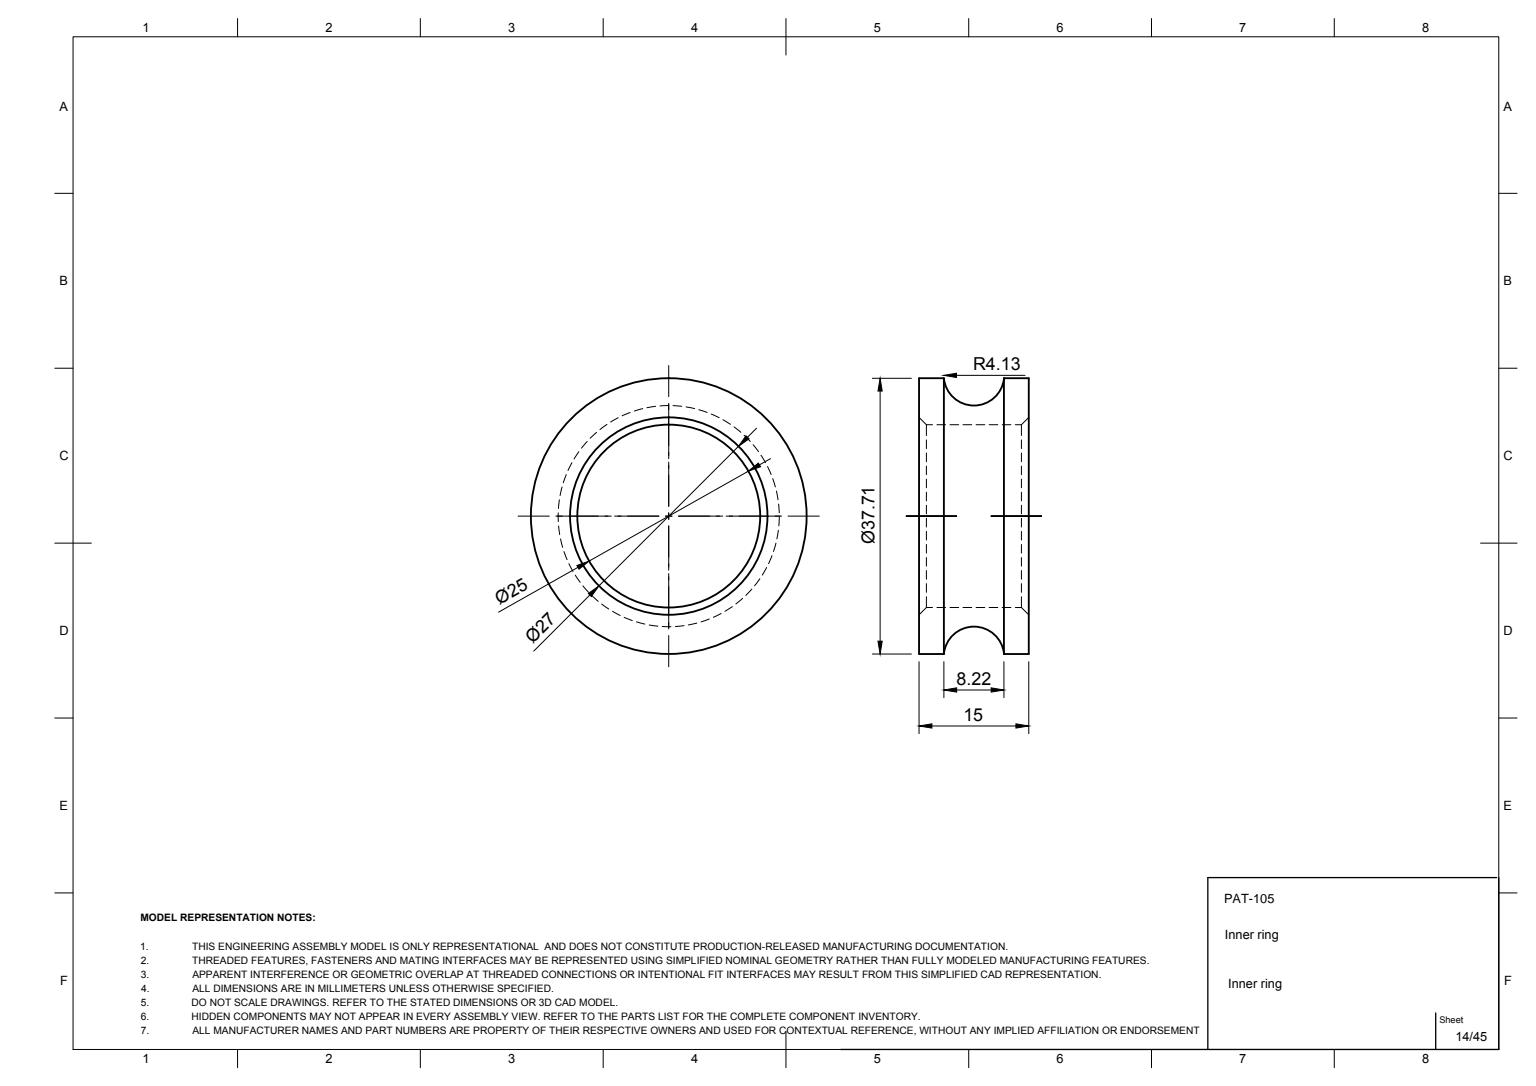
ISO-10303-21;
HEADER;
/* Generated by software containing ST-Developer
 * from STEP Tools, Inc. (www.steptools.com) 
 */

FILE_DESCRIPTION(
/* description */ ('Torque wrench calibration arm'),
/* implementation_level */ '2;1');

FILE_NAME(
/* name */ 'Inner ring.step',
/* time_stamp */ '2026-10-28T03:24:52-07:00',
/* author */ (''),
/* organization */ (''),
/* preprocessor_version */ 'ST-DEVELOPER v20.2',
/* originating_system */ 'Autodesk Translation Framework v15.17.0.0',
/* authorisation */ '');

FILE_SCHEMA (('AUTOMOTIVE_DESIGN { 1 0 10303 214 3 1 1 }'));
ENDSEC;

DATA;
#10=MECHANICAL_DESIGN_GEOMETRIC_PRESENTATION_REPRESENTATION('',(#433),#12783);
#327=CONICAL_SURFACE('',#7170,1.3,0.785398163397449);
#328=CONICAL_SURFACE('',#7177,1.3,0.785398163397449);
#348=TOROIDAL_SURFACE('',#7159,1.925,0.412776);
#359=SHAPE_REPRESENTATION_RELATIONSHIP('SRR','None',#12941,#396);
#396=ADVANCED_BREP_SHAPE_REPRESENTATION('',(#487),#12750);
#433=STYLED_ITEM('',(#13212),#487);
#487=MANIFOLD_SOLID_BREP('Body1',#6502);
#583=FACE_BOUND('',#1427,.T.);
#584=FACE_BOUND('',#1430,.T.);
#710=PLANE('',#7172);
#711=PLANE('',#7175);
#975=FACE_OUTER_BOUND('',#1422,.T.);
#976=FACE_OUTER_BOUND('',#1423,.T.);
#977=FACE_OUTER_BOUND('',#1424,.T.);
#978=FACE_OUTER_BOUND('',#1425,.T.);
#979=FACE_OUTER_BOUND('',#1426,.T.);
#980=FACE_OUTER_BOUND('',#1428,.T.);
#981=FACE_OUTER_BOUND('',#1429,.T.);
#982=FACE_OUTER_BOUND('',#1431,.T.);
#1422=EDGE_LOOP('',(#4795,#4796,#4797,#4798,#4799,#4800));
#1423=EDGE_LOOP('',(#4801,#4802,#4803,#4804,#4805));
#1424=EDGE_LOOP('',(#4806,#4807,#4808,#4809));
#1425=EDGE_LOOP('',(#4810,#4811,#4812,#4813));
#1426=EDGE_LOOP('',(#4814));
#1427=EDGE_LOOP('',(#4815));
#1428=EDGE_LOOP('',(#4816,#4817,#4818,#4819,#4820));
#1429=EDGE_LOOP('',(#4821));
#1430=EDGE_LOOP('',(#4822));
#1431=EDGE_LOOP('',(#4823,#4824,#4825,#4826));
#1920=LINE('',#10418,#2335);
#1921=LINE('',#10424,#2336);
#1922=LINE('',#10428,#2337);
#1923=LINE('',#10434,#2338);
#1924=LINE('',#10439,#2339);
#2335=VECTOR('',#8356,1.88531);
#2336=VECTOR('',#8363,1.25);
#2337=VECTOR('',#8368,1.3);
#2338=VECTOR('',#8377,1.88531);
#2339=VECTOR('',#8384,1.3);
#2704=CIRCLE('',#7160,1.88531);
#2705=CIRCLE('',#7161,1.88531);
#2706=CIRCLE('',#7162,0.412776);
#2707=CIRCLE('',#7163,1.88531);
#2708=CIRCLE('',#7164,1.88531);
#2709=CIRCLE('',#7166,1.88531);
#2710=CIRCLE('',#7168,1.25);
#2711=CIRCLE('',#7169,1.25);
#2712=CIRCLE('',#7171,1.35);
#2713=CIRCLE('',#7174,1.88531);
#2714=CIRCLE('',#7176,1.35);
#3119=VERTEX_POINT('',#10407);
#3120=VERTEX_POINT('',#10408);
#3121=VERTEX_POINT('',#10411);
#3122=VERTEX_POINT('',#10413);
#3123=VERTEX_POINT('',#10417);
#3124=VERTEX_POINT('',#10421);
#3125=VERTEX_POINT('',#10423);
#3126=VERTEX_POINT('',#10427);
#3127=VERTEX_POINT('',#10432);
#3128=VERTEX_POINT('',#10436);
#3755=EDGE_CURVE('',#3119,#3120,#2704,.T.);
#3756=EDGE_CURVE('',#3120,#3119,#2705,.T.);
#3757=EDGE_CURVE('',#3120,#3121,#2706,.T.);
#3758=EDGE_CURVE('',#3122,#3121,#2707,.T.);
#3759=EDGE_CURVE('',#3121,#3122,#2708,.T.);
#3760=EDGE_CURVE('',#3122,#3123,#1920,.T.);
#3761=EDGE_CURVE('',#3123,#3123,#2709,.T.);
#3762=EDGE_CURVE('',#3124,#3124,#2710,.T.);
#3763=EDGE_CURVE('',#3124,#3125,#1921,.T.);
#3764=EDGE_CURVE('',#3125,#3125,#2711,.T.);
#3765=EDGE_CURVE('',#3125,#3126,#1922,.T.);
#3766=EDGE_CURVE('',#3126,#3126,#2712,.T.);
#3767=EDGE_CURVE('',#3127,#3127,#2713,.T.);
#3768=EDGE_CURVE('',#3127,#3119,#1923,.T.);
#3769=EDGE_CURVE('',#3128,#3128,#2714,.T.);
#3770=EDGE_CURVE('',#3128,#3124,#1924,.T.);
#4795=ORIENTED_EDGE('',*,*,#3755,.F.);
#4796=ORIENTED_EDGE('',*,*,#3756,.F.);
#4797=ORIENTED_EDGE('',*,*,#3757,.T.);
#4798=ORIENTED_EDGE('',*,*,#3758,.F.);
#4799=ORIENTED_EDGE('',*,*,#3759,.F.);
#4800=ORIENTED_EDGE('',*,*,#3757,.F.);
#4801=ORIENTED_EDGE('',*,*,#3758,.T.);
#4802=ORIENTED_EDGE('',*,*,#3759,.T.);
#4803=ORIENTED_EDGE('',*,*,#3760,.T.);
#4804=ORIENTED_EDGE('',*,*,#3761,.T.);
#4805=ORIENTED_EDGE('',*,*,#3760,.F.);
#4806=ORIENTED_EDGE('',*,*,#3762,.T.);
#4807=ORIENTED_EDGE('',*,*,#3763,.T.);
#4808=ORIENTED_EDGE('',*,*,#3764,.F.);
#4809=ORIENTED_EDGE('',*,*,#3763,.F.);
#4810=ORIENTED_EDGE('',*,*,#3764,.T.);
#4811=ORIENTED_EDGE('',*,*,#3765,.T.);
#4812=ORIENTED_EDGE('',*,*,#3766,.F.);
#4813=ORIENTED_EDGE('',*,*,#3765,.F.);
#4814=ORIENTED_EDGE('',*,*,#3761,.F.);
#4815=ORIENTED_EDGE('',*,*,#3766,.T.);
#4816=ORIENTED_EDGE('',*,*,#3767,.F.);
#4817=ORIENTED_EDGE('',*,*,#3768,.T.);
#4818=ORIENTED_EDGE('',*,*,#3755,.T.);
#4819=ORIENTED_EDGE('',*,*,#3756,.T.);
#4820=ORIENTED_EDGE('',*,*,#3768,.F.);
#4821=ORIENTED_EDGE('',*,*,#3767,.T.);
#4822=ORIENTED_EDGE('',*,*,#3769,.F.);
#4823=ORIENTED_EDGE('',*,*,#3769,.T.);
#4824=ORIENTED_EDGE('',*,*,#3770,.T.);
#4825=ORIENTED_EDGE('',*,*,#3762,.F.);
#4826=ORIENTED_EDGE('',*,*,#3770,.F.);
#6029=CYLINDRICAL_SURFACE('',#7165,1.88531);
#6030=CYLINDRICAL_SURFACE('',#7167,1.25);
#6031=CYLINDRICAL_SURFACE('',#7173,1.88531);
#6200=ADVANCED_FACE('',(#975),#348,.F.);
#6201=ADVANCED_FACE('',(#976),#6029,.T.);
#6202=ADVANCED_FACE('',(#977),#6030,.F.);
#6203=ADVANCED_FACE('',(#978),#327,.F.);
#6204=ADVANCED_FACE('',(#979,#583),#710,.T.);
#6205=ADVANCED_FACE('',(#980),#6031,.T.);
#6206=ADVANCED_FACE('',(#981,#584),#711,.T.);
#6207=ADVANCED_FACE('',(#982),#328,.F.);
#6502=CLOSED_SHELL('',(#6200,#6201,#6202,#6203,#6204,#6205,#6206,#6207));
#7158=AXIS2_PLACEMENT_3D('',#10405,#8340,#8341);
#7159=AXIS2_PLACEMENT_3D('',#10406,#8342,#8343);
#7160=AXIS2_PLACEMENT_3D('',#10409,#8344,#8345);
#7161=AXIS2_PLACEMENT_3D('',#10410,#8346,#8347);
#7162=AXIS2_PLACEMENT_3D('',#10412,#8348,#8349);
#7163=AXIS2_PLACEMENT_3D('',#10414,#8350,#8351);
#7164=AXIS2_PLACEMENT_3D('',#10415,#8352,#8353);
#7165=AXIS2_PLACEMENT_3D('',#10416,#8354,#8355);
#7166=AXIS2_PLACEMENT_3D('',#10419,#8357,#8358);
#7167=AXIS2_PLACEMENT_3D('',#10420,#8359,#8360);
#7168=AXIS2_PLACEMENT_3D('',#10422,#8361,#8362);
#7169=AXIS2_PLACEMENT_3D('',#10425,#8364,#8365);
#7170=AXIS2_PLACEMENT_3D('',#10426,#8366,#8367);
#7171=AXIS2_PLACEMENT_3D('',#10429,#8369,#8370);
#7172=AXIS2_PLACEMENT_3D('',#10430,#8371,#8372);
#7173=AXIS2_PLACEMENT_3D('',#10431,#8373,#8374);
#7174=AXIS2_PLACEMENT_3D('',#10433,#8375,#8376);
#7175=AXIS2_PLACEMENT_3D('',#10435,#8378,#8379);
#7176=AXIS2_PLACEMENT_3D('',#10437,#8380,#8381);
#7177=AXIS2_PLACEMENT_3D('',#10438,#8382,#8383);
#8340=DIRECTION('axis',(0.,0.,1.));
#8341=DIRECTION('refdir',(1.,0.,0.));
#8342=DIRECTION('center_axis',(0.,-1.,0.));
#8343=DIRECTION('ref_axis',(0.,0.,-1.));
#8344=DIRECTION('center_axis',(0.,-1.,0.));
#8345=DIRECTION('ref_axis',(1.,0.,0.));
#8346=DIRECTION('center_axis',(0.,-1.,0.));
#8347=DIRECTION('ref_axis',(1.,0.,0.));
#8348=DIRECTION('center_axis',(1.,0.,1.22464679914735E-16));
#8349=DIRECTION('ref_axis',(-1.22464679914735E-16,0.,1.));
#8350=DIRECTION('center_axis',(0.,1.,0.));
#8351=DIRECTION('ref_axis',(1.,0.,0.));
#8352=DIRECTION('center_axis',(0.,1.,0.));
#8353=DIRECTION('ref_axis',(1.,0.,0.));
#8354=DIRECTION('center_axis',(0.,-1.,0.));
#8355=DIRECTION('ref_axis',(1.,0.,0.));
#8356=DIRECTION('',(0.,1.,0.));
#8357=DIRECTION('center_axis',(0.,-1.,0.));
#8358=DIRECTION('ref_axis',(1.,0.,0.));
#8359=DIRECTION('center_axis',(0.,-1.,0.));
#8360=DIRECTION('ref_axis',(1.,0.,0.));
#8361=DIRECTION('center_axis',(0.,-1.,0.));
#8362=DIRECTION('ref_axis',(1.,0.,0.));
#8363=DIRECTION('',(0.,1.,0.));
#8364=DIRECTION('center_axis',(0.,-1.,0.));
#8365=DIRECTION('ref_axis',(1.,0.,0.));
#8366=DIRECTION('center_axis',(0.,1.,0.));
#8367=DIRECTION('ref_axis',(1.,0.,0.));
#8368=DIRECTION('',(-0.707106781186548,0.707106781186547,-8.65956056235494E-17));
#8369=DIRECTION('center_axis',(0.,-1.,0.));
#8370=DIRECTION('ref_axis',(1.,0.,0.));
#8371=DIRECTION('center_axis',(0.,1.,0.));
#8372=DIRECTION('ref_axis',(0.,0.,1.));
#8373=DIRECTION('center_axis',(0.,-1.,0.));
#8374=DIRECTION('ref_axis',(1.,0.,0.));
#8375=DIRECTION('center_axis',(0.,-1.,0.));
#8376=DIRECTION('ref_axis',(1.,0.,0.));
#8377=DIRECTION('',(0.,1.,0.));
#8378=DIRECTION('center_axis',(0.,-1.,0.));
#8379=DIRECTION('ref_axis',(0.,0.,-1.));
#8380=DIRECTION('center_axis',(0.,-1.,0.));
#8381=DIRECTION('ref_axis',(1.,0.,0.));
#8382=DIRECTION('center_axis',(0.,-1.,0.));
#8383=DIRECTION('ref_axis',(1.,0.,0.));
#8384=DIRECTION('',(0.707106781186548,0.707106781186547,8.65956056235494E-17));
#10405=CARTESIAN_POINT('',(0.,0.,0.));
#10406=CARTESIAN_POINT('Origin',(0.,0.,0.));
#10407=CARTESIAN_POINT('',(-1.88531,-0.410863395882378,-2.3088388569005E-16));
#10408=CARTESIAN_POINT('',(-2.3088388569005E-16,-0.410863395882378,1.88531));
#10409=CARTESIAN_POINT('Origin',(0.,-0.410863395882378,0.));
#10410=CARTESIAN_POINT('Origin',(0.,-0.410863395882378,0.));
#10411=CARTESIAN_POINT('',(-2.3088388569005E-16,0.410863395882378,1.88531));
#10412=CARTESIAN_POINT('Origin',(-2.35744508835865E-16,0.,1.925));
#10413=CARTESIAN_POINT('',(-1.88531,0.410863395882378,2.3088388569005E-16));
#10414=CARTESIAN_POINT('Origin',(0.,0.410863395882378,0.));
#10415=CARTESIAN_POINT('Origin',(0.,0.410863395882378,0.));
#10416=CARTESIAN_POINT('Origin',(0.,0.,0.));
#10417=CARTESIAN_POINT('',(-1.88531,0.75,-2.3088388569005E-16));
#10418=CARTESIAN_POINT('',(-1.88531,0.,-2.3088388569005E-16));
#10419=CARTESIAN_POINT('Origin',(0.,0.75,0.));
#10420=CARTESIAN_POINT('Origin',(0.,0.,0.));
#10421=CARTESIAN_POINT('',(-1.25,-0.65,-1.53080849893419E-16));
#10422=CARTESIAN_POINT('Origin',(0.,-0.65,0.));
#10423=CARTESIAN_POINT('',(-1.25,0.65,-1.53080849893419E-16));
#10424=CARTESIAN_POINT('',(-1.25,0.,-1.53080849893419E-16));
#10425=CARTESIAN_POINT('Origin',(0.,0.65,0.));
#10426=CARTESIAN_POINT('Origin',(0.,0.7,0.));
#10427=CARTESIAN_POINT('',(-1.35,0.75,-1.65327317884893E-16));
#10428=CARTESIAN_POINT('',(-1.3,0.7,-1.59204083889156E-16));
#10429=CARTESIAN_POINT('Origin',(0.,0.75,0.));
#10430=CARTESIAN_POINT('Origin',(1.88531,0.75,0.));
#10431=CARTESIAN_POINT('Origin',(0.,0.,0.));
#10432=CARTESIAN_POINT('',(-1.88531,-0.75,-2.3088388569005E-16));
#10433=CARTESIAN_POINT('Origin',(0.,-0.75,0.));
#10434=CARTESIAN_POINT('',(-1.88531,0.,-2.3088388569005E-16));
#10435=CARTESIAN_POINT('Origin',(1.35,-0.75,0.));
#10436=CARTESIAN_POINT('',(-1.35,-0.75,-1.65327317884893E-16));
#10437=CARTESIAN_POINT('Origin',(0.,-0.75,0.));
#10438=CARTESIAN_POINT('Origin',(0.,-0.7,0.));
#10439=CARTESIAN_POINT('',(-1.3,-0.7,-1.59204083889156E-16));
#12706=UNCERTAINTY_MEASURE_WITH_UNIT(LENGTH_MEASURE(0.001),#12784,
'DISTANCE_ACCURACY_VALUE',
'Maximum model space distance between geometric entities at asserted c
onnectivities');
#12739=UNCERTAINTY_MEASURE_WITH_UNIT(LENGTH_MEASURE(0.001),#12784,
'DISTANCE_ACCURACY_VALUE',
'Maximum model space distance between geometric entities at asserted c
onnectivities');
#12750=(
GEOMETRIC_REPRESENTATION_CONTEXT(3)
GLOBAL_UNCERTAINTY_ASSIGNED_CONTEXT((#12706))
GLOBAL_UNIT_ASSIGNED_CONTEXT((#12784,#12786,#12787))
REPRESENTATION_CONTEXT('','3D')
);
#12783=(
GEOMETRIC_REPRESENTATION_CONTEXT(3)
GLOBAL_UNCERTAINTY_ASSIGNED_CONTEXT((#12739))
GLOBAL_UNIT_ASSIGNED_CONTEXT((#12784,#12786,#12787))
REPRESENTATION_CONTEXT('','3D')
);
#12784=(
LENGTH_UNIT()
NAMED_UNIT(*)
SI_UNIT(.CENTI.,.METRE.)
);
#12786=(
NAMED_UNIT(*)
PLANE_ANGLE_UNIT()
SI_UNIT($,.RADIAN.)
);
#12787=(
NAMED_UNIT(*)
SI_UNIT($,.STERADIAN.)
SOLID_ANGLE_UNIT()
);
#12798=SHAPE_DEFINITION_REPRESENTATION(#12841,#12941);
#12841=PRODUCT_DEFINITION_SHAPE('',$,#12985);
#12941=SHAPE_REPRESENTATION('',(#7158),#12750);
#12974=PRODUCT_DEFINITION_CONTEXT('part definition',#13105,'design');
#12985=PRODUCT_DEFINITION('Inner ring','Inner ring',#13028,#12974);
#13028=PRODUCT_DEFINITION_FORMATION('',$,#13117);
#13105=APPLICATION_CONTEXT(
'Core Data for Automotive Mechanical Design Process');
#13106=PRODUCT_CONTEXT('part definition',#13105,'mechanical');
#13117=PRODUCT('Inner ring','Inner ring','Inner ring',(#13106));
#13206=COLOUR_RGB('Grey',0.48,0.52,0.57);
#13207=FILL_AREA_STYLE_COLOUR('',#13206);
#13208=FILL_AREA_STYLE('',(#13207));
#13209=SURFACE_STYLE_FILL_AREA(#13208);
#13210=SURFACE_SIDE_STYLE('',(#13209));
#13211=SURFACE_STYLE_USAGE(.BOTH.,#13210);
#13212=PRESENTATION_STYLE_ASSIGNMENT((#13211));
ENDSEC;
END-ISO-10303-21;
